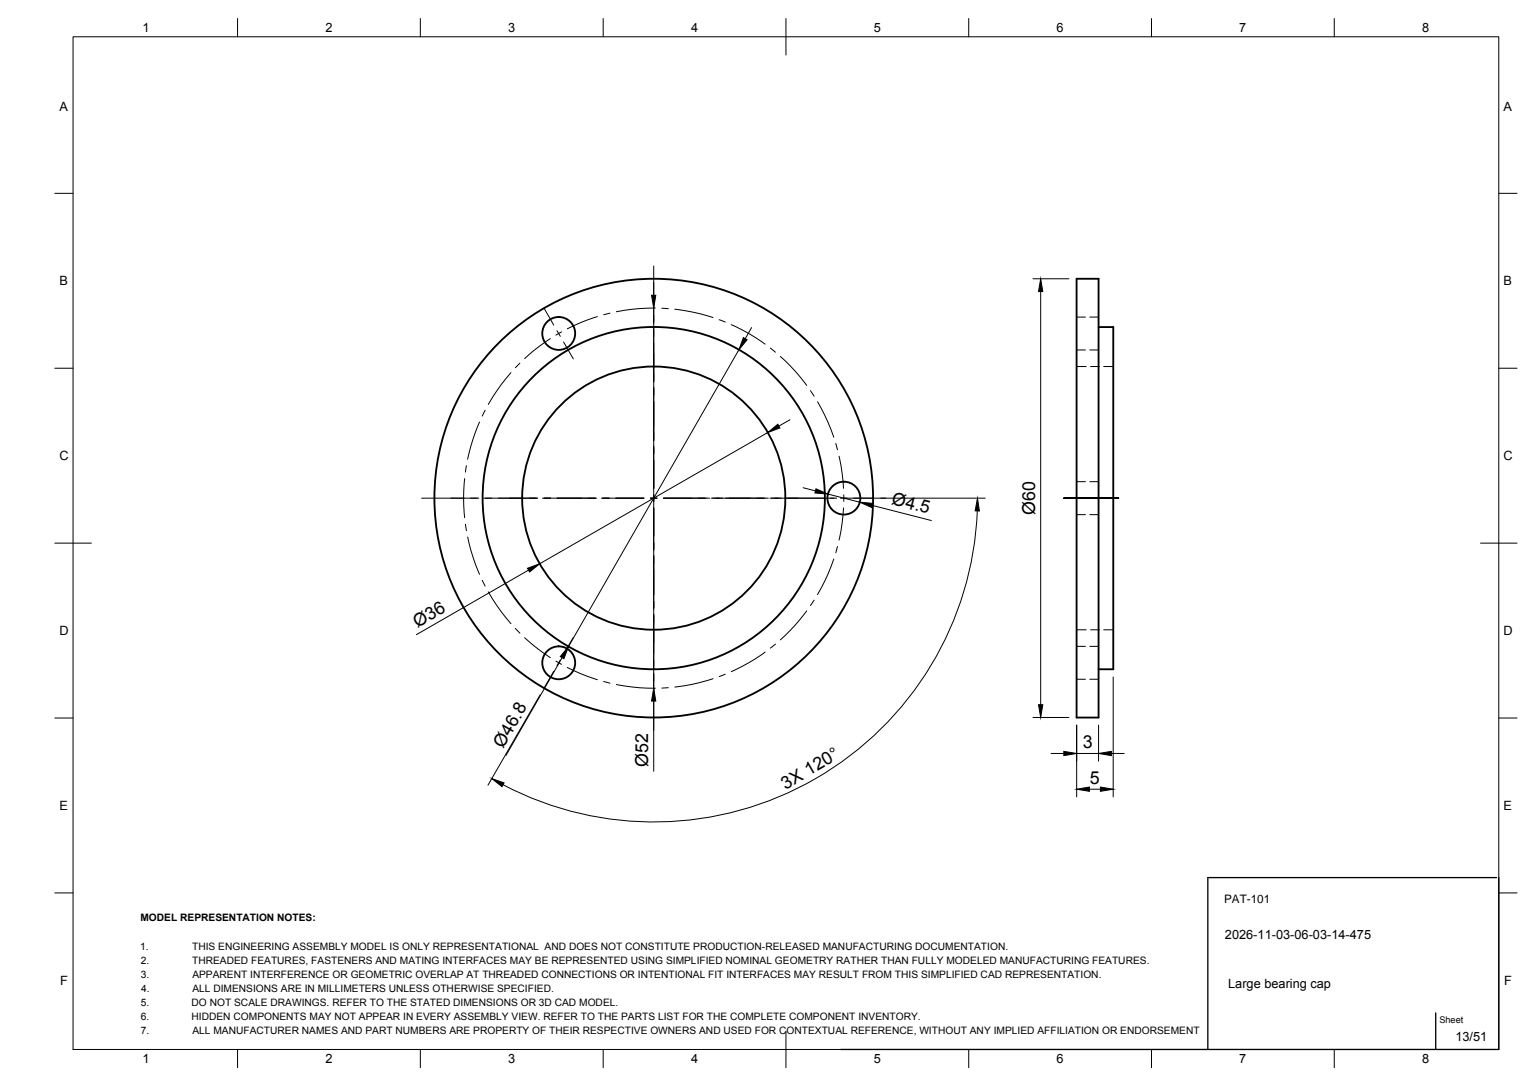
ISO-10303-21;
HEADER;
/* Generated by software containing ST-Developer
 * from STEP Tools, Inc. (www.steptools.com) 
 */

FILE_DESCRIPTION(
/* description */ ('Spur gear reduction stage 2-1 on bearing plates'),
/* implementation_level */ '2;1');

FILE_NAME(
/* name */ 'Large bearing cap.step',
/* time_stamp */ '2026-10-28T03:22:07-07:00',
/* author */ (''),
/* organization */ (''),
/* preprocessor_version */ 'ST-DEVELOPER v20.2',
/* originating_system */ 'Autodesk Translation Framework v15.17.0.0',
/* authorisation */ '');

FILE_SCHEMA (('AUTOMOTIVE_DESIGN { 1 0 10303 214 3 1 1 }'));
ENDSEC;

DATA;
#10=MECHANICAL_DESIGN_GEOMETRIC_PRESENTATION_REPRESENTATION('',(#955),#53909);
#869=SHAPE_REPRESENTATION_RELATIONSHIP('SRR','None',#54096,#912);
#912=ADVANCED_BREP_SHAPE_REPRESENTATION('',(#1013),#53870);
#955=STYLED_ITEM('',(#54397),#1013);
#1013=MANIFOLD_SOLID_BREP('Body1',#11279);
#1149=FACE_BOUND('',#2348,.T.);
#1150=FACE_BOUND('',#2352,.T.);
#1151=FACE_BOUND('',#2353,.T.);
#1152=FACE_BOUND('',#2354,.T.);
#1153=FACE_BOUND('',#2355,.T.);
#1154=FACE_BOUND('',#2357,.T.);
#1155=FACE_BOUND('',#2358,.T.);
#1156=FACE_BOUND('',#2359,.T.);
#1157=FACE_BOUND('',#2360,.T.);
#1283=PLANE('',#12048);
#1284=PLANE('',#12055);
#1285=PLANE('',#12056);
#1606=FACE_OUTER_BOUND('',#2343,.T.);
#1607=FACE_OUTER_BOUND('',#2344,.T.);
#1608=FACE_OUTER_BOUND('',#2345,.T.);
#1609=FACE_OUTER_BOUND('',#2346,.T.);
#1610=FACE_OUTER_BOUND('',#2347,.T.);
#1611=FACE_OUTER_BOUND('',#2349,.T.);
#1612=FACE_OUTER_BOUND('',#2350,.T.);
#1613=FACE_OUTER_BOUND('',#2351,.T.);
#1614=FACE_OUTER_BOUND('',#2356,.T.);
#2343=EDGE_LOOP('',(#7772,#7773,#7774,#7775));
#2344=EDGE_LOOP('',(#7776,#7777,#7778,#7779));
#2345=EDGE_LOOP('',(#7780,#7781,#7782,#7783));
#2346=EDGE_LOOP('',(#7784,#7785,#7786,#7787));
#2347=EDGE_LOOP('',(#7788));
#2348=EDGE_LOOP('',(#7789));
#2349=EDGE_LOOP('',(#7790,#7791,#7792,#7793));
#2350=EDGE_LOOP('',(#7794,#7795,#7796,#7797));
#2351=EDGE_LOOP('',(#7798));
#2352=EDGE_LOOP('',(#7799));
#2353=EDGE_LOOP('',(#7800));
#2354=EDGE_LOOP('',(#7801));
#2355=EDGE_LOOP('',(#7802));
#2356=EDGE_LOOP('',(#7803));
#2357=EDGE_LOOP('',(#7804));
#2358=EDGE_LOOP('',(#7805));
#2359=EDGE_LOOP('',(#7806));
#2360=EDGE_LOOP('',(#7807));
#3071=LINE('',#16443,#3712);
#3072=LINE('',#16449,#3713);
#3073=LINE('',#16455,#3714);
#3074=LINE('',#16461,#3715);
#3075=LINE('',#16468,#3716);
#3076=LINE('',#16474,#3717);
#3712=VECTOR('',#13540,0.225);
#3713=VECTOR('',#13547,0.225);
#3714=VECTOR('',#13554,0.225);
#3715=VECTOR('',#13561,2.34);
#3716=VECTOR('',#13570,1.8);
#3717=VECTOR('',#13577,3.);
#4375=CIRCLE('',#12037,0.225);
#4376=CIRCLE('',#12038,0.225);
#4377=CIRCLE('',#12040,0.225);
#4378=CIRCLE('',#12041,0.225);
#4379=CIRCLE('',#12043,0.225);
#4380=CIRCLE('',#12044,0.225);
#4381=CIRCLE('',#12046,2.34);
#4382=CIRCLE('',#12047,2.34);
#4383=CIRCLE('',#12049,1.8);
#4384=CIRCLE('',#12051,1.8);
#4385=CIRCLE('',#12053,3.);
#4386=CIRCLE('',#12054,3.);
#4924=VERTEX_POINT('',#16440);
#4925=VERTEX_POINT('',#16442);
#4926=VERTEX_POINT('',#16446);
#4927=VERTEX_POINT('',#16448);
#4928=VERTEX_POINT('',#16452);
#4929=VERTEX_POINT('',#16454);
#4930=VERTEX_POINT('',#16458);
#4931=VERTEX_POINT('',#16460);
#4932=VERTEX_POINT('',#16464);
#4933=VERTEX_POINT('',#16467);
#4934=VERTEX_POINT('',#16471);
#4935=VERTEX_POINT('',#16473);
#6028=EDGE_CURVE('',#4924,#4924,#4375,.T.);
#6029=EDGE_CURVE('',#4924,#4925,#3071,.T.);
#6030=EDGE_CURVE('',#4925,#4925,#4376,.T.);
#6031=EDGE_CURVE('',#4926,#4926,#4377,.T.);
#6032=EDGE_CURVE('',#4926,#4927,#3072,.T.);
#6033=EDGE_CURVE('',#4927,#4927,#4378,.T.);
#6034=EDGE_CURVE('',#4928,#4928,#4379,.T.);
#6035=EDGE_CURVE('',#4928,#4929,#3073,.T.);
#6036=EDGE_CURVE('',#4929,#4929,#4380,.T.);
#6037=EDGE_CURVE('',#4930,#4930,#4381,.T.);
#6038=EDGE_CURVE('',#4930,#4931,#3074,.T.);
#6039=EDGE_CURVE('',#4931,#4931,#4382,.T.);
#6040=EDGE_CURVE('',#4932,#4932,#4383,.T.);
#6041=EDGE_CURVE('',#4932,#4933,#3075,.T.);
#6042=EDGE_CURVE('',#4933,#4933,#4384,.T.);
#6043=EDGE_CURVE('',#4934,#4934,#4385,.T.);
#6044=EDGE_CURVE('',#4934,#4935,#3076,.T.);
#6045=EDGE_CURVE('',#4935,#4935,#4386,.T.);
#7772=ORIENTED_EDGE('',*,*,#6028,.F.);
#7773=ORIENTED_EDGE('',*,*,#6029,.T.);
#7774=ORIENTED_EDGE('',*,*,#6030,.F.);
#7775=ORIENTED_EDGE('',*,*,#6029,.F.);
#7776=ORIENTED_EDGE('',*,*,#6031,.F.);
#7777=ORIENTED_EDGE('',*,*,#6032,.T.);
#7778=ORIENTED_EDGE('',*,*,#6033,.F.);
#7779=ORIENTED_EDGE('',*,*,#6032,.F.);
#7780=ORIENTED_EDGE('',*,*,#6034,.F.);
#7781=ORIENTED_EDGE('',*,*,#6035,.T.);
#7782=ORIENTED_EDGE('',*,*,#6036,.F.);
#7783=ORIENTED_EDGE('',*,*,#6035,.F.);
#7784=ORIENTED_EDGE('',*,*,#6037,.F.);
#7785=ORIENTED_EDGE('',*,*,#6038,.T.);
#7786=ORIENTED_EDGE('',*,*,#6039,.F.);
#7787=ORIENTED_EDGE('',*,*,#6038,.F.);
#7788=ORIENTED_EDGE('',*,*,#6037,.T.);
#7789=ORIENTED_EDGE('',*,*,#6040,.T.);
#7790=ORIENTED_EDGE('',*,*,#6040,.F.);
#7791=ORIENTED_EDGE('',*,*,#6041,.T.);
#7792=ORIENTED_EDGE('',*,*,#6042,.T.);
#7793=ORIENTED_EDGE('',*,*,#6041,.F.);
#7794=ORIENTED_EDGE('',*,*,#6043,.F.);
#7795=ORIENTED_EDGE('',*,*,#6044,.T.);
#7796=ORIENTED_EDGE('',*,*,#6045,.T.);
#7797=ORIENTED_EDGE('',*,*,#6044,.F.);
#7798=ORIENTED_EDGE('',*,*,#6043,.T.);
#7799=ORIENTED_EDGE('',*,*,#6030,.T.);
#7800=ORIENTED_EDGE('',*,*,#6033,.T.);
#7801=ORIENTED_EDGE('',*,*,#6036,.T.);
#7802=ORIENTED_EDGE('',*,*,#6039,.T.);
#7803=ORIENTED_EDGE('',*,*,#6045,.F.);
#7804=ORIENTED_EDGE('',*,*,#6028,.T.);
#7805=ORIENTED_EDGE('',*,*,#6031,.T.);
#7806=ORIENTED_EDGE('',*,*,#6034,.T.);
#7807=ORIENTED_EDGE('',*,*,#6042,.F.);
#10478=CYLINDRICAL_SURFACE('',#12036,0.225);
#10479=CYLINDRICAL_SURFACE('',#12039,0.225);
#10480=CYLINDRICAL_SURFACE('',#12042,0.225);
#10481=CYLINDRICAL_SURFACE('',#12045,2.34);
#10482=CYLINDRICAL_SURFACE('',#12050,1.8);
#10483=CYLINDRICAL_SURFACE('',#12052,3.);
#10726=ADVANCED_FACE('',(#1606),#10478,.F.);
#10727=ADVANCED_FACE('',(#1607),#10479,.F.);
#10728=ADVANCED_FACE('',(#1608),#10480,.F.);
#10729=ADVANCED_FACE('',(#1609),#10481,.T.);
#10730=ADVANCED_FACE('',(#1610,#1149),#1283,.T.);
#10731=ADVANCED_FACE('',(#1611),#10482,.F.);
#10732=ADVANCED_FACE('',(#1612),#10483,.T.);
#10733=ADVANCED_FACE('',(#1613,#1150,#1151,#1152,#1153),#1284,.T.);
#10734=ADVANCED_FACE('',(#1614,#1154,#1155,#1156,#1157),#1285,.F.);
#11279=CLOSED_SHELL('',(#10726,#10727,#10728,#10729,#10730,#10731,#10732,
#10733,#10734));
#12035=AXIS2_PLACEMENT_3D('',#16438,#13534,#13535);
#12036=AXIS2_PLACEMENT_3D('',#16439,#13536,#13537);
#12037=AXIS2_PLACEMENT_3D('',#16441,#13538,#13539);
#12038=AXIS2_PLACEMENT_3D('',#16444,#13541,#13542);
#12039=AXIS2_PLACEMENT_3D('',#16445,#13543,#13544);
#12040=AXIS2_PLACEMENT_3D('',#16447,#13545,#13546);
#12041=AXIS2_PLACEMENT_3D('',#16450,#13548,#13549);
#12042=AXIS2_PLACEMENT_3D('',#16451,#13550,#13551);
#12043=AXIS2_PLACEMENT_3D('',#16453,#13552,#13553);
#12044=AXIS2_PLACEMENT_3D('',#16456,#13555,#13556);
#12045=AXIS2_PLACEMENT_3D('',#16457,#13557,#13558);
#12046=AXIS2_PLACEMENT_3D('',#16459,#13559,#13560);
#12047=AXIS2_PLACEMENT_3D('',#16462,#13562,#13563);
#12048=AXIS2_PLACEMENT_3D('',#16463,#13564,#13565);
#12049=AXIS2_PLACEMENT_3D('',#16465,#13566,#13567);
#12050=AXIS2_PLACEMENT_3D('',#16466,#13568,#13569);
#12051=AXIS2_PLACEMENT_3D('',#16469,#13571,#13572);
#12052=AXIS2_PLACEMENT_3D('',#16470,#13573,#13574);
#12053=AXIS2_PLACEMENT_3D('',#16472,#13575,#13576);
#12054=AXIS2_PLACEMENT_3D('',#16475,#13578,#13579);
#12055=AXIS2_PLACEMENT_3D('',#16476,#13580,#13581);
#12056=AXIS2_PLACEMENT_3D('',#16477,#13582,#13583);
#13534=DIRECTION('axis',(0.,0.,1.));
#13535=DIRECTION('refdir',(1.,0.,0.));
#13536=DIRECTION('center_axis',(0.,1.,0.));
#13537=DIRECTION('ref_axis',(1.,0.,0.));
#13538=DIRECTION('center_axis',(0.,1.,0.));
#13539=DIRECTION('ref_axis',(1.,0.,0.));
#13540=DIRECTION('',(0.,1.,0.));
#13541=DIRECTION('center_axis',(0.,-1.,0.));
#13542=DIRECTION('ref_axis',(1.,0.,0.));
#13543=DIRECTION('center_axis',(0.,1.,0.));
#13544=DIRECTION('ref_axis',(1.,0.,0.));
#13545=DIRECTION('center_axis',(0.,1.,0.));
#13546=DIRECTION('ref_axis',(1.,0.,0.));
#13547=DIRECTION('',(0.,1.,0.));
#13548=DIRECTION('center_axis',(0.,-1.,0.));
#13549=DIRECTION('ref_axis',(1.,0.,0.));
#13550=DIRECTION('center_axis',(0.,1.,0.));
#13551=DIRECTION('ref_axis',(1.,0.,0.));
#13552=DIRECTION('center_axis',(0.,1.,0.));
#13553=DIRECTION('ref_axis',(1.,0.,0.));
#13554=DIRECTION('',(0.,1.,0.));
#13555=DIRECTION('center_axis',(0.,-1.,0.));
#13556=DIRECTION('ref_axis',(1.,0.,0.));
#13557=DIRECTION('center_axis',(0.,1.,0.));
#13558=DIRECTION('ref_axis',(1.,0.,0.));
#13559=DIRECTION('center_axis',(0.,1.,0.));
#13560=DIRECTION('ref_axis',(1.,0.,0.));
#13561=DIRECTION('',(0.,-1.,0.));
#13562=DIRECTION('center_axis',(0.,-1.,0.));
#13563=DIRECTION('ref_axis',(1.,0.,0.));
#13564=DIRECTION('center_axis',(0.,1.,0.));
#13565=DIRECTION('ref_axis',(1.,0.,0.));
#13566=DIRECTION('center_axis',(0.,-1.,0.));
#13567=DIRECTION('ref_axis',(1.,0.,0.));
#13568=DIRECTION('center_axis',(0.,1.,0.));
#13569=DIRECTION('ref_axis',(1.,0.,0.));
#13570=DIRECTION('',(0.,-1.,0.));
#13571=DIRECTION('center_axis',(0.,-1.,0.));
#13572=DIRECTION('ref_axis',(1.,0.,0.));
#13573=DIRECTION('center_axis',(0.,1.,0.));
#13574=DIRECTION('ref_axis',(1.,0.,0.));
#13575=DIRECTION('center_axis',(0.,1.,0.));
#13576=DIRECTION('ref_axis',(1.,0.,0.));
#13577=DIRECTION('',(0.,-1.,0.));
#13578=DIRECTION('center_axis',(0.,1.,0.));
#13579=DIRECTION('ref_axis',(1.,0.,0.));
#13580=DIRECTION('center_axis',(0.,1.,0.));
#13581=DIRECTION('ref_axis',(1.,0.,0.));
#13582=DIRECTION('center_axis',(0.,1.,0.));
#13583=DIRECTION('ref_axis',(1.,0.,0.));
#16438=CARTESIAN_POINT('',(0.,0.,0.));
#16439=CARTESIAN_POINT('Origin',(6.,-4.8,7.6));
#16440=CARTESIAN_POINT('',(5.775,-4.7,7.6));
#16441=CARTESIAN_POINT('Origin',(6.,-4.7,7.6));
#16442=CARTESIAN_POINT('',(5.775,-4.4,7.6));
#16443=CARTESIAN_POINT('',(5.775,-4.8,7.6));
#16444=CARTESIAN_POINT('Origin',(6.,-4.4,7.6));
#16445=CARTESIAN_POINT('Origin',(3.74833395016046,-4.8,3.7));
#16446=CARTESIAN_POINT('',(3.52333395016046,-4.7,3.7));
#16447=CARTESIAN_POINT('Origin',(3.74833395016046,-4.7,3.7));
#16448=CARTESIAN_POINT('',(3.52333395016046,-4.4,3.7));
#16449=CARTESIAN_POINT('',(3.52333395016046,-4.8,3.7));
#16450=CARTESIAN_POINT('Origin',(3.74833395016046,-4.4,3.7));
#16451=CARTESIAN_POINT('Origin',(8.25166604983954,-4.8,3.7));
#16452=CARTESIAN_POINT('',(8.02666604983954,-4.7,3.7));
#16453=CARTESIAN_POINT('Origin',(8.25166604983954,-4.7,3.7));
#16454=CARTESIAN_POINT('',(8.02666604983954,-4.4,3.7));
#16455=CARTESIAN_POINT('',(8.02666604983954,-4.8,3.7));
#16456=CARTESIAN_POINT('Origin',(8.25166604983954,-4.4,3.7));
#16457=CARTESIAN_POINT('Origin',(6.,-4.4,5.));
#16458=CARTESIAN_POINT('',(3.66,-4.2,5.));
#16459=CARTESIAN_POINT('Origin',(6.,-4.2,5.));
#16460=CARTESIAN_POINT('',(3.66,-4.4,5.));
#16461=CARTESIAN_POINT('',(3.66,-4.4,5.));
#16462=CARTESIAN_POINT('Origin',(6.,-4.4,5.));
#16463=CARTESIAN_POINT('Origin',(6.,-4.2,5.));
#16464=CARTESIAN_POINT('',(4.2,-4.2,5.));
#16465=CARTESIAN_POINT('Origin',(6.,-4.2,5.));
#16466=CARTESIAN_POINT('Origin',(6.,-4.7,5.));
#16467=CARTESIAN_POINT('',(4.2,-4.7,5.));
#16468=CARTESIAN_POINT('',(4.2,-4.7,5.));
#16469=CARTESIAN_POINT('Origin',(6.,-4.7,5.));
#16470=CARTESIAN_POINT('Origin',(6.,-4.7,5.));
#16471=CARTESIAN_POINT('',(3.,-4.4,5.));
#16472=CARTESIAN_POINT('Origin',(6.,-4.4,5.));
#16473=CARTESIAN_POINT('',(3.,-4.7,5.));
#16474=CARTESIAN_POINT('',(3.,-4.7,5.));
#16475=CARTESIAN_POINT('Origin',(6.,-4.7,5.));
#16476=CARTESIAN_POINT('Origin',(6.,-4.4,5.));
#16477=CARTESIAN_POINT('Origin',(6.,-4.7,5.));
#53820=UNCERTAINTY_MEASURE_WITH_UNIT(LENGTH_MEASURE(0.001),#53910,
'DISTANCE_ACCURACY_VALUE',
'Maximum model space distance between geometric entities at asserted c
onnectivities');
#53859=UNCERTAINTY_MEASURE_WITH_UNIT(LENGTH_MEASURE(0.001),#53910,
'DISTANCE_ACCURACY_VALUE',
'Maximum model space distance between geometric entities at asserted c
onnectivities');
#53870=(
GEOMETRIC_REPRESENTATION_CONTEXT(3)
GLOBAL_UNCERTAINTY_ASSIGNED_CONTEXT((#53820))
GLOBAL_UNIT_ASSIGNED_CONTEXT((#53910,#53912,#53913))
REPRESENTATION_CONTEXT('','3D')
);
#53909=(
GEOMETRIC_REPRESENTATION_CONTEXT(3)
GLOBAL_UNCERTAINTY_ASSIGNED_CONTEXT((#53859))
GLOBAL_UNIT_ASSIGNED_CONTEXT((#53910,#53912,#53913))
REPRESENTATION_CONTEXT('','3D')
);
#53910=(
LENGTH_UNIT()
NAMED_UNIT(*)
SI_UNIT(.CENTI.,.METRE.)
);
#53912=(
NAMED_UNIT(*)
PLANE_ANGLE_UNIT()
SI_UNIT($,.RADIAN.)
);
#53913=(
NAMED_UNIT(*)
SI_UNIT($,.STERADIAN.)
SOLID_ANGLE_UNIT()
);
#53924=SHAPE_DEFINITION_REPRESENTATION(#53973,#54096);
#53973=PRODUCT_DEFINITION_SHAPE('',$,#54146);
#54096=SHAPE_REPRESENTATION('',(#12035),#53870);
#54135=PRODUCT_DEFINITION_CONTEXT('part definition',#54284,'design');
#54146=PRODUCT_DEFINITION('Large bearing cap','Large bearing cap',#54195,
#54135);
#54195=PRODUCT_DEFINITION_FORMATION('',$,#54296);
#54284=APPLICATION_CONTEXT(
'Core Data for Automotive Mechanical Design Process');
#54285=PRODUCT_CONTEXT('part definition',#54284,'mechanical');
#54296=PRODUCT('Large bearing cap','Large bearing cap',
'Large bearing cap',(#54285));
#54391=COLOUR_RGB('Grey',0.48,0.52,0.57);
#54392=FILL_AREA_STYLE_COLOUR('',#54391);
#54393=FILL_AREA_STYLE('',(#54392));
#54394=SURFACE_STYLE_FILL_AREA(#54393);
#54395=SURFACE_SIDE_STYLE('',(#54394));
#54396=SURFACE_STYLE_USAGE(.BOTH.,#54395);
#54397=PRESENTATION_STYLE_ASSIGNMENT((#54396));
ENDSEC;
END-ISO-10303-21;
